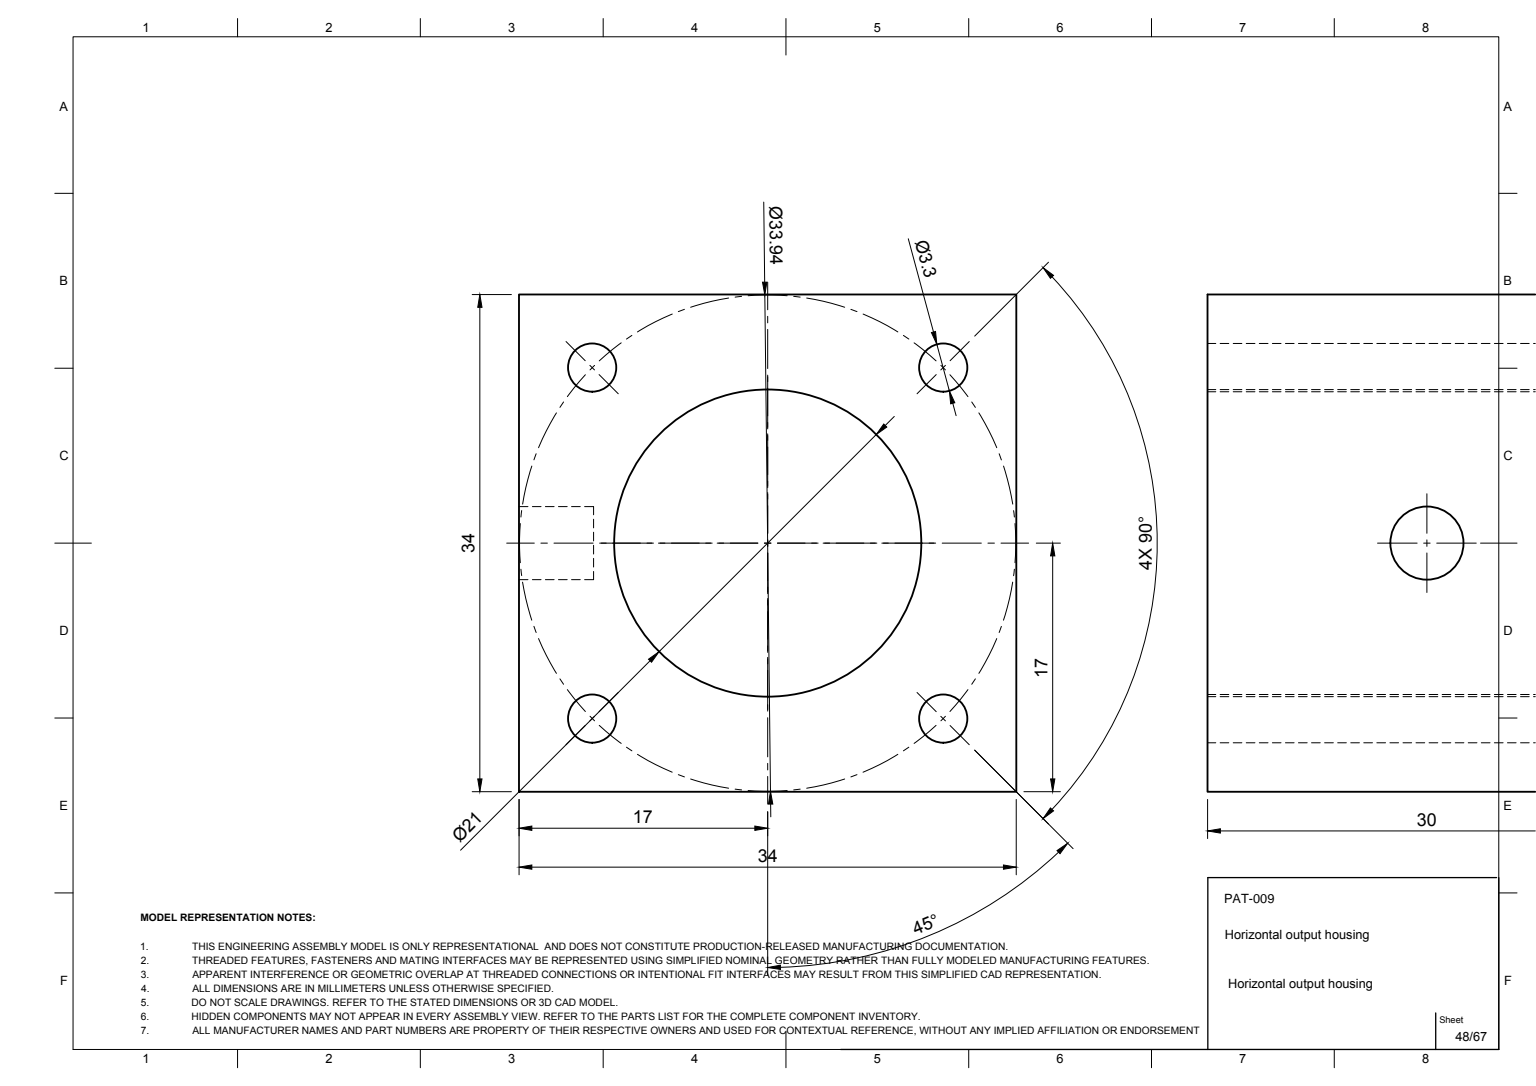
ISO-10303-21;
HEADER;
/* Generated by software containing ST-Developer
 * from STEP Tools, Inc. (www.steptools.com) 
 */

FILE_DESCRIPTION(
/* description */ ('Bell-crank linkage with push rods'),
/* implementation_level */ '2;1');

FILE_NAME(
/* name */ 'Horizontal output housing.step',
/* time_stamp */ '2026-10-28T03:25:15-07:00',
/* author */ (''),
/* organization */ (''),
/* preprocessor_version */ 'ST-DEVELOPER v20.2',
/* originating_system */ 'Autodesk Translation Framework v15.17.0.0',
/* authorisation */ '');

FILE_SCHEMA (('AUTOMOTIVE_DESIGN { 1 0 10303 214 3 1 1 }'));
ENDSEC;

DATA;
#10=MECHANICAL_DESIGN_GEOMETRIC_PRESENTATION_REPRESENTATION('',(#649),#16678);
#533=SHAPE_REPRESENTATION_RELATIONSHIP('SRR','None',#16954,#587);
#587=ADVANCED_BREP_SHAPE_REPRESENTATION('',(#709),#16659);
#649=STYLED_ITEM('',(#17270),#709);
#709=MANIFOLD_SOLID_BREP('Body1',#8841);
#874=FACE_BOUND('',#2296,.T.);
#875=FACE_BOUND('',#2297,.T.);
#876=FACE_BOUND('',#2298,.T.);
#877=FACE_BOUND('',#2299,.T.);
#878=FACE_BOUND('',#2300,.T.);
#879=FACE_BOUND('',#2303,.T.);
#880=FACE_BOUND('',#2304,.T.);
#881=FACE_BOUND('',#2305,.T.);
#882=FACE_BOUND('',#2306,.T.);
#883=FACE_BOUND('',#2307,.T.);
#884=FACE_BOUND('',#2309,.T.);
#1159=PLANE('',#10239);
#1160=PLANE('',#10255);
#1161=PLANE('',#10256);
#1162=PLANE('',#10257);
#1163=PLANE('',#10258);
#1164=PLANE('',#10259);
#1165=PLANE('',#10260);
#1616=FACE_OUTER_BOUND('',#2287,.T.);
#1617=FACE_OUTER_BOUND('',#2288,.T.);
#1618=FACE_OUTER_BOUND('',#2289,.T.);
#1619=FACE_OUTER_BOUND('',#2290,.T.);
#1620=FACE_OUTER_BOUND('',#2291,.T.);
#1621=FACE_OUTER_BOUND('',#2292,.T.);
#1622=FACE_OUTER_BOUND('',#2293,.T.);
#1623=FACE_OUTER_BOUND('',#2294,.T.);
#1624=FACE_OUTER_BOUND('',#2295,.T.);
#1625=FACE_OUTER_BOUND('',#2301,.T.);
#1626=FACE_OUTER_BOUND('',#2302,.T.);
#1627=FACE_OUTER_BOUND('',#2308,.T.);
#1628=FACE_OUTER_BOUND('',#2310,.T.);
#2287=EDGE_LOOP('',(#7455,#7456,#7457,#7458));
#2288=EDGE_LOOP('',(#7459));
#2289=EDGE_LOOP('',(#7460,#7461,#7462,#7463));
#2290=EDGE_LOOP('',(#7464,#7465,#7466,#7467));
#2291=EDGE_LOOP('',(#7468,#7469,#7470,#7471));
#2292=EDGE_LOOP('',(#7472,#7473,#7474,#7475));
#2293=EDGE_LOOP('',(#7476,#7477,#7478,#7479));
#2294=EDGE_LOOP('',(#7480,#7481,#7482,#7483));
#2295=EDGE_LOOP('',(#7484,#7485,#7486,#7487));
#2296=EDGE_LOOP('',(#7488));
#2297=EDGE_LOOP('',(#7489));
#2298=EDGE_LOOP('',(#7490));
#2299=EDGE_LOOP('',(#7491));
#2300=EDGE_LOOP('',(#7492));
#2301=EDGE_LOOP('',(#7493,#7494,#7495,#7496));
#2302=EDGE_LOOP('',(#7497,#7498,#7499,#7500));
#2303=EDGE_LOOP('',(#7501));
#2304=EDGE_LOOP('',(#7502));
#2305=EDGE_LOOP('',(#7503));
#2306=EDGE_LOOP('',(#7504));
#2307=EDGE_LOOP('',(#7505));
#2308=EDGE_LOOP('',(#7506,#7507,#7508,#7509));
#2309=EDGE_LOOP('',(#7510));
#2310=EDGE_LOOP('',(#7511,#7512,#7513,#7514));
#2908=LINE('',#15785,#3457);
#2909=LINE('',#15792,#3458);
#2910=LINE('',#15798,#3459);
#2911=LINE('',#15804,#3460);
#2912=LINE('',#15810,#3461);
#2913=LINE('',#15816,#3462);
#2914=LINE('',#15821,#3463);
#2915=LINE('',#15823,#3464);
#2916=LINE('',#15825,#3465);
#2917=LINE('',#15826,#3466);
#2918=LINE('',#15829,#3467);
#2919=LINE('',#15831,#3468);
#2920=LINE('',#15832,#3469);
#2921=LINE('',#15835,#3470);
#2922=LINE('',#15837,#3471);
#2923=LINE('',#15838,#3472);
#2924=LINE('',#15840,#3473);
#2925=LINE('',#15841,#3474);
#3457=VECTOR('',#12574,0.25);
#3458=VECTOR('',#12583,0.165);
#3459=VECTOR('',#12590,0.165);
#3460=VECTOR('',#12597,0.165);
#3461=VECTOR('',#12604,0.165);
#3462=VECTOR('',#12611,1.05);
#3463=VECTOR('',#12616,1.);
#3464=VECTOR('',#12617,1.);
#3465=VECTOR('',#12618,1.);
#3466=VECTOR('',#12619,1.);
#3467=VECTOR('',#12622,1.);
#3468=VECTOR('',#12623,1.);
#3469=VECTOR('',#12624,1.);
#3470=VECTOR('',#12627,1.);
#3471=VECTOR('',#12628,1.);
#3472=VECTOR('',#12629,1.);
#3473=VECTOR('',#12632,1.);
#3474=VECTOR('',#12633,1.);
#3987=CIRCLE('',#10237,0.25);
#3988=CIRCLE('',#10238,0.25);
#3989=CIRCLE('',#10241,0.165);
#3990=CIRCLE('',#10242,0.165);
#3991=CIRCLE('',#10244,0.165);
#3992=CIRCLE('',#10245,0.165);
#3993=CIRCLE('',#10247,0.165);
#3994=CIRCLE('',#10248,0.165);
#3995=CIRCLE('',#10250,0.165);
#3996=CIRCLE('',#10251,0.165);
#3997=CIRCLE('',#10253,1.05);
#3998=CIRCLE('',#10254,1.05);
#4630=VERTEX_POINT('',#15782);
#4631=VERTEX_POINT('',#15784);
#4632=VERTEX_POINT('',#15789);
#4633=VERTEX_POINT('',#15791);
#4634=VERTEX_POINT('',#15795);
#4635=VERTEX_POINT('',#15797);
#4636=VERTEX_POINT('',#15801);
#4637=VERTEX_POINT('',#15803);
#4638=VERTEX_POINT('',#15807);
#4639=VERTEX_POINT('',#15809);
#4640=VERTEX_POINT('',#15813);
#4641=VERTEX_POINT('',#15815);
#4642=VERTEX_POINT('',#15819);
#4643=VERTEX_POINT('',#15820);
#4644=VERTEX_POINT('',#15822);
#4645=VERTEX_POINT('',#15824);
#4646=VERTEX_POINT('',#15828);
#4647=VERTEX_POINT('',#15830);
#4648=VERTEX_POINT('',#15834);
#4649=VERTEX_POINT('',#15836);
#5605=EDGE_CURVE('',#4630,#4630,#3987,.T.);
#5606=EDGE_CURVE('',#4630,#4631,#2908,.T.);
#5607=EDGE_CURVE('',#4631,#4631,#3988,.T.);
#5608=EDGE_CURVE('',#4632,#4632,#3989,.T.);
#5609=EDGE_CURVE('',#4632,#4633,#2909,.T.);
#5610=EDGE_CURVE('',#4633,#4633,#3990,.T.);
#5611=EDGE_CURVE('',#4634,#4634,#3991,.T.);
#5612=EDGE_CURVE('',#4634,#4635,#2910,.T.);
#5613=EDGE_CURVE('',#4635,#4635,#3992,.T.);
#5614=EDGE_CURVE('',#4636,#4636,#3993,.T.);
#5615=EDGE_CURVE('',#4636,#4637,#2911,.T.);
#5616=EDGE_CURVE('',#4637,#4637,#3994,.T.);
#5617=EDGE_CURVE('',#4638,#4638,#3995,.T.);
#5618=EDGE_CURVE('',#4638,#4639,#2912,.T.);
#5619=EDGE_CURVE('',#4639,#4639,#3996,.T.);
#5620=EDGE_CURVE('',#4640,#4640,#3997,.T.);
#5621=EDGE_CURVE('',#4640,#4641,#2913,.T.);
#5622=EDGE_CURVE('',#4641,#4641,#3998,.T.);
#5623=EDGE_CURVE('',#4642,#4643,#2914,.T.);
#5624=EDGE_CURVE('',#4643,#4644,#2915,.T.);
#5625=EDGE_CURVE('',#4645,#4644,#2916,.T.);
#5626=EDGE_CURVE('',#4642,#4645,#2917,.T.);
#5627=EDGE_CURVE('',#4646,#4642,#2918,.T.);
#5628=EDGE_CURVE('',#4647,#4645,#2919,.T.);
#5629=EDGE_CURVE('',#4646,#4647,#2920,.T.);
#5630=EDGE_CURVE('',#4648,#4646,#2921,.T.);
#5631=EDGE_CURVE('',#4649,#4647,#2922,.T.);
#5632=EDGE_CURVE('',#4648,#4649,#2923,.T.);
#5633=EDGE_CURVE('',#4643,#4648,#2924,.T.);
#5634=EDGE_CURVE('',#4644,#4649,#2925,.T.);
#7455=ORIENTED_EDGE('',*,*,#5605,.F.);
#7456=ORIENTED_EDGE('',*,*,#5606,.T.);
#7457=ORIENTED_EDGE('',*,*,#5607,.F.);
#7458=ORIENTED_EDGE('',*,*,#5606,.F.);
#7459=ORIENTED_EDGE('',*,*,#5605,.T.);
#7460=ORIENTED_EDGE('',*,*,#5608,.F.);
#7461=ORIENTED_EDGE('',*,*,#5609,.T.);
#7462=ORIENTED_EDGE('',*,*,#5610,.F.);
#7463=ORIENTED_EDGE('',*,*,#5609,.F.);
#7464=ORIENTED_EDGE('',*,*,#5611,.F.);
#7465=ORIENTED_EDGE('',*,*,#5612,.T.);
#7466=ORIENTED_EDGE('',*,*,#5613,.F.);
#7467=ORIENTED_EDGE('',*,*,#5612,.F.);
#7468=ORIENTED_EDGE('',*,*,#5614,.F.);
#7469=ORIENTED_EDGE('',*,*,#5615,.T.);
#7470=ORIENTED_EDGE('',*,*,#5616,.F.);
#7471=ORIENTED_EDGE('',*,*,#5615,.F.);
#7472=ORIENTED_EDGE('',*,*,#5617,.F.);
#7473=ORIENTED_EDGE('',*,*,#5618,.T.);
#7474=ORIENTED_EDGE('',*,*,#5619,.F.);
#7475=ORIENTED_EDGE('',*,*,#5618,.F.);
#7476=ORIENTED_EDGE('',*,*,#5620,.F.);
#7477=ORIENTED_EDGE('',*,*,#5621,.T.);
#7478=ORIENTED_EDGE('',*,*,#5622,.F.);
#7479=ORIENTED_EDGE('',*,*,#5621,.F.);
#7480=ORIENTED_EDGE('',*,*,#5623,.T.);
#7481=ORIENTED_EDGE('',*,*,#5624,.T.);
#7482=ORIENTED_EDGE('',*,*,#5625,.F.);
#7483=ORIENTED_EDGE('',*,*,#5626,.F.);
#7484=ORIENTED_EDGE('',*,*,#5627,.T.);
#7485=ORIENTED_EDGE('',*,*,#5626,.T.);
#7486=ORIENTED_EDGE('',*,*,#5628,.F.);
#7487=ORIENTED_EDGE('',*,*,#5629,.F.);
#7488=ORIENTED_EDGE('',*,*,#5622,.T.);
#7489=ORIENTED_EDGE('',*,*,#5619,.T.);
#7490=ORIENTED_EDGE('',*,*,#5616,.T.);
#7491=ORIENTED_EDGE('',*,*,#5613,.T.);
#7492=ORIENTED_EDGE('',*,*,#5610,.T.);
#7493=ORIENTED_EDGE('',*,*,#5630,.T.);
#7494=ORIENTED_EDGE('',*,*,#5629,.T.);
#7495=ORIENTED_EDGE('',*,*,#5631,.F.);
#7496=ORIENTED_EDGE('',*,*,#5632,.F.);
#7497=ORIENTED_EDGE('',*,*,#5633,.T.);
#7498=ORIENTED_EDGE('',*,*,#5632,.T.);
#7499=ORIENTED_EDGE('',*,*,#5634,.F.);
#7500=ORIENTED_EDGE('',*,*,#5624,.F.);
#7501=ORIENTED_EDGE('',*,*,#5620,.T.);
#7502=ORIENTED_EDGE('',*,*,#5617,.T.);
#7503=ORIENTED_EDGE('',*,*,#5614,.T.);
#7504=ORIENTED_EDGE('',*,*,#5611,.T.);
#7505=ORIENTED_EDGE('',*,*,#5608,.T.);
#7506=ORIENTED_EDGE('',*,*,#5634,.T.);
#7507=ORIENTED_EDGE('',*,*,#5631,.T.);
#7508=ORIENTED_EDGE('',*,*,#5628,.T.);
#7509=ORIENTED_EDGE('',*,*,#5625,.T.);
#7510=ORIENTED_EDGE('',*,*,#5607,.T.);
#7511=ORIENTED_EDGE('',*,*,#5633,.F.);
#7512=ORIENTED_EDGE('',*,*,#5623,.F.);
#7513=ORIENTED_EDGE('',*,*,#5627,.F.);
#7514=ORIENTED_EDGE('',*,*,#5630,.F.);
#8210=CYLINDRICAL_SURFACE('',#10236,0.25);
#8211=CYLINDRICAL_SURFACE('',#10240,0.165);
#8212=CYLINDRICAL_SURFACE('',#10243,0.165);
#8213=CYLINDRICAL_SURFACE('',#10246,0.165);
#8214=CYLINDRICAL_SURFACE('',#10249,0.165);
#8215=CYLINDRICAL_SURFACE('',#10252,1.05);
#8641=ADVANCED_FACE('',(#1616),#8210,.F.);
#8642=ADVANCED_FACE('',(#1617),#1159,.T.);
#8643=ADVANCED_FACE('',(#1618),#8211,.F.);
#8644=ADVANCED_FACE('',(#1619),#8212,.F.);
#8645=ADVANCED_FACE('',(#1620),#8213,.F.);
#8646=ADVANCED_FACE('',(#1621),#8214,.F.);
#8647=ADVANCED_FACE('',(#1622),#8215,.F.);
#8648=ADVANCED_FACE('',(#1623),#1160,.T.);
#8649=ADVANCED_FACE('',(#1624,#874,#875,#876,#877,#878),#1161,.T.);
#8650=ADVANCED_FACE('',(#1625),#1162,.T.);
#8651=ADVANCED_FACE('',(#1626,#879,#880,#881,#882,#883),#1163,.T.);
#8652=ADVANCED_FACE('',(#1627,#884),#1164,.T.);
#8653=ADVANCED_FACE('',(#1628),#1165,.F.);
#8841=CLOSED_SHELL('',(#8641,#8642,#8643,#8644,#8645,#8646,#8647,#8648,
#8649,#8650,#8651,#8652,#8653));
#10235=AXIS2_PLACEMENT_3D('',#15780,#12568,#12569);
#10236=AXIS2_PLACEMENT_3D('',#15781,#12570,#12571);
#10237=AXIS2_PLACEMENT_3D('',#15783,#12572,#12573);
#10238=AXIS2_PLACEMENT_3D('',#15786,#12575,#12576);
#10239=AXIS2_PLACEMENT_3D('',#15787,#12577,#12578);
#10240=AXIS2_PLACEMENT_3D('',#15788,#12579,#12580);
#10241=AXIS2_PLACEMENT_3D('',#15790,#12581,#12582);
#10242=AXIS2_PLACEMENT_3D('',#15793,#12584,#12585);
#10243=AXIS2_PLACEMENT_3D('',#15794,#12586,#12587);
#10244=AXIS2_PLACEMENT_3D('',#15796,#12588,#12589);
#10245=AXIS2_PLACEMENT_3D('',#15799,#12591,#12592);
#10246=AXIS2_PLACEMENT_3D('',#15800,#12593,#12594);
#10247=AXIS2_PLACEMENT_3D('',#15802,#12595,#12596);
#10248=AXIS2_PLACEMENT_3D('',#15805,#12598,#12599);
#10249=AXIS2_PLACEMENT_3D('',#15806,#12600,#12601);
#10250=AXIS2_PLACEMENT_3D('',#15808,#12602,#12603);
#10251=AXIS2_PLACEMENT_3D('',#15811,#12605,#12606);
#10252=AXIS2_PLACEMENT_3D('',#15812,#12607,#12608);
#10253=AXIS2_PLACEMENT_3D('',#15814,#12609,#12610);
#10254=AXIS2_PLACEMENT_3D('',#15817,#12612,#12613);
#10255=AXIS2_PLACEMENT_3D('',#15818,#12614,#12615);
#10256=AXIS2_PLACEMENT_3D('',#15827,#12620,#12621);
#10257=AXIS2_PLACEMENT_3D('',#15833,#12625,#12626);
#10258=AXIS2_PLACEMENT_3D('',#15839,#12630,#12631);
#10259=AXIS2_PLACEMENT_3D('',#15842,#12634,#12635);
#10260=AXIS2_PLACEMENT_3D('',#15843,#12636,#12637);
#12568=DIRECTION('axis',(0.,0.,1.));
#12569=DIRECTION('refdir',(1.,0.,0.));
#12570=DIRECTION('center_axis',(0.,0.,1.));
#12571=DIRECTION('ref_axis',(1.,0.,0.));
#12572=DIRECTION('center_axis',(0.,0.,1.));
#12573=DIRECTION('ref_axis',(1.,0.,0.));
#12574=DIRECTION('',(0.,0.,1.));
#12575=DIRECTION('center_axis',(0.,0.,-1.));
#12576=DIRECTION('ref_axis',(1.,0.,0.));
#12577=DIRECTION('center_axis',(0.,0.,1.));
#12578=DIRECTION('ref_axis',(1.,0.,0.));
#12579=DIRECTION('center_axis',(1.,0.,0.));
#12580=DIRECTION('ref_axis',(0.,0.,-1.));
#12581=DIRECTION('center_axis',(1.,0.,0.));
#12582=DIRECTION('ref_axis',(0.,0.,-1.));
#12583=DIRECTION('',(1.,0.,0.));
#12584=DIRECTION('center_axis',(-1.,0.,0.));
#12585=DIRECTION('ref_axis',(0.,0.,-1.));
#12586=DIRECTION('center_axis',(1.,0.,0.));
#12587=DIRECTION('ref_axis',(0.,0.,-1.));
#12588=DIRECTION('center_axis',(1.,0.,0.));
#12589=DIRECTION('ref_axis',(0.,0.,-1.));
#12590=DIRECTION('',(1.,0.,0.));
#12591=DIRECTION('center_axis',(-1.,0.,0.));
#12592=DIRECTION('ref_axis',(0.,0.,-1.));
#12593=DIRECTION('center_axis',(1.,0.,0.));
#12594=DIRECTION('ref_axis',(0.,0.,-1.));
#12595=DIRECTION('center_axis',(1.,0.,0.));
#12596=DIRECTION('ref_axis',(0.,0.,-1.));
#12597=DIRECTION('',(1.,0.,0.));
#12598=DIRECTION('center_axis',(-1.,0.,0.));
#12599=DIRECTION('ref_axis',(0.,0.,-1.));
#12600=DIRECTION('center_axis',(1.,0.,0.));
#12601=DIRECTION('ref_axis',(0.,0.,-1.));
#12602=DIRECTION('center_axis',(1.,0.,0.));
#12603=DIRECTION('ref_axis',(0.,0.,-1.));
#12604=DIRECTION('',(1.,0.,0.));
#12605=DIRECTION('center_axis',(-1.,0.,0.));
#12606=DIRECTION('ref_axis',(0.,0.,-1.));
#12607=DIRECTION('center_axis',(1.,0.,0.));
#12608=DIRECTION('ref_axis',(0.,0.,-1.));
#12609=DIRECTION('center_axis',(1.,0.,0.));
#12610=DIRECTION('ref_axis',(0.,0.,-1.));
#12611=DIRECTION('',(1.,0.,0.));
#12612=DIRECTION('center_axis',(-1.,0.,0.));
#12613=DIRECTION('ref_axis',(0.,0.,-1.));
#12614=DIRECTION('center_axis',(0.,1.,0.));
#12615=DIRECTION('ref_axis',(-1.,0.,0.));
#12616=DIRECTION('',(-1.,0.,0.));
#12617=DIRECTION('',(0.,0.,1.));
#12618=DIRECTION('',(-1.,0.,0.));
#12619=DIRECTION('',(0.,0.,1.));
#12620=DIRECTION('center_axis',(1.,0.,0.));
#12621=DIRECTION('ref_axis',(0.,1.,0.));
#12622=DIRECTION('',(0.,1.,0.));
#12623=DIRECTION('',(0.,1.,0.));
#12624=DIRECTION('',(0.,0.,1.));
#12625=DIRECTION('center_axis',(0.,-1.,0.));
#12626=DIRECTION('ref_axis',(1.,0.,0.));
#12627=DIRECTION('',(1.,0.,0.));
#12628=DIRECTION('',(1.,0.,0.));
#12629=DIRECTION('',(0.,0.,1.));
#12630=DIRECTION('center_axis',(-1.,0.,0.));
#12631=DIRECTION('ref_axis',(0.,-1.,0.));
#12632=DIRECTION('',(0.,-1.,0.));
#12633=DIRECTION('',(0.,-1.,0.));
#12634=DIRECTION('center_axis',(0.,0.,1.));
#12635=DIRECTION('ref_axis',(1.,0.,0.));
#12636=DIRECTION('center_axis',(0.,0.,1.));
#12637=DIRECTION('ref_axis',(1.,0.,0.));
#15780=CARTESIAN_POINT('',(0.,0.,0.));
#15781=CARTESIAN_POINT('Origin',(10.,2.,5.19));
#15782=CARTESIAN_POINT('',(9.75,2.,5.19));
#15783=CARTESIAN_POINT('Origin',(10.,2.,5.19));
#15784=CARTESIAN_POINT('',(9.75,2.,5.7));
#15785=CARTESIAN_POINT('',(9.75,2.,5.19));
#15786=CARTESIAN_POINT('Origin',(10.,2.,5.7));
#15787=CARTESIAN_POINT('Origin',(10.,2.,5.19));
#15788=CARTESIAN_POINT('Origin',(8.4,3.2,2.8));
#15789=CARTESIAN_POINT('',(8.5,3.2,2.965));
#15790=CARTESIAN_POINT('Origin',(8.5,3.2,2.8));
#15791=CARTESIAN_POINT('',(11.5,3.2,2.965));
#15792=CARTESIAN_POINT('',(8.4,3.2,2.965));
#15793=CARTESIAN_POINT('Origin',(11.5,3.2,2.8));
#15794=CARTESIAN_POINT('Origin',(8.4,0.8,5.2));
#15795=CARTESIAN_POINT('',(8.5,0.8,5.365));
#15796=CARTESIAN_POINT('Origin',(8.5,0.8,5.2));
#15797=CARTESIAN_POINT('',(11.5,0.8,5.365));
#15798=CARTESIAN_POINT('',(8.4,0.8,5.365));
#15799=CARTESIAN_POINT('Origin',(11.5,0.8,5.2));
#15800=CARTESIAN_POINT('Origin',(8.4,0.8,2.8));
#15801=CARTESIAN_POINT('',(8.5,0.8,2.965));
#15802=CARTESIAN_POINT('Origin',(8.5,0.8,2.8));
#15803=CARTESIAN_POINT('',(11.5,0.8,2.965));
#15804=CARTESIAN_POINT('',(8.4,0.8,2.965));
#15805=CARTESIAN_POINT('Origin',(11.5,0.8,2.8));
#15806=CARTESIAN_POINT('Origin',(8.4,3.2,5.2));
#15807=CARTESIAN_POINT('',(8.5,3.2,5.365));
#15808=CARTESIAN_POINT('Origin',(8.5,3.2,5.2));
#15809=CARTESIAN_POINT('',(11.5,3.2,5.365));
#15810=CARTESIAN_POINT('',(8.4,3.2,5.365));
#15811=CARTESIAN_POINT('Origin',(11.5,3.2,5.2));
#15812=CARTESIAN_POINT('Origin',(8.4,2.,4.));
#15813=CARTESIAN_POINT('',(8.5,2.,5.05));
#15814=CARTESIAN_POINT('Origin',(8.5,2.,4.));
#15815=CARTESIAN_POINT('',(11.5,2.,5.05));
#15816=CARTESIAN_POINT('',(8.4,2.,5.05));
#15817=CARTESIAN_POINT('Origin',(11.5,2.,4.));
#15818=CARTESIAN_POINT('Origin',(11.5,3.7,2.3));
#15819=CARTESIAN_POINT('',(11.5,3.7,2.3));
#15820=CARTESIAN_POINT('',(8.5,3.7,2.3));
#15821=CARTESIAN_POINT('',(11.5,3.7,2.3));
#15822=CARTESIAN_POINT('',(8.5,3.7,5.7));
#15823=CARTESIAN_POINT('',(8.5,3.7,2.3));
#15824=CARTESIAN_POINT('',(11.5,3.7,5.7));
#15825=CARTESIAN_POINT('',(11.5,3.7,5.7));
#15826=CARTESIAN_POINT('',(11.5,3.7,2.3));
#15827=CARTESIAN_POINT('Origin',(11.5,0.3,2.3));
#15828=CARTESIAN_POINT('',(11.5,0.3,2.3));
#15829=CARTESIAN_POINT('',(11.5,0.3,2.3));
#15830=CARTESIAN_POINT('',(11.5,0.3,5.7));
#15831=CARTESIAN_POINT('',(11.5,0.3,5.7));
#15832=CARTESIAN_POINT('',(11.5,0.3,2.3));
#15833=CARTESIAN_POINT('Origin',(8.5,0.3,2.3));
#15834=CARTESIAN_POINT('',(8.5,0.3,2.3));
#15835=CARTESIAN_POINT('',(8.5,0.3,2.3));
#15836=CARTESIAN_POINT('',(8.5,0.3,5.7));
#15837=CARTESIAN_POINT('',(8.5,0.3,5.7));
#15838=CARTESIAN_POINT('',(8.5,0.3,2.3));
#15839=CARTESIAN_POINT('Origin',(8.5,3.7,2.3));
#15840=CARTESIAN_POINT('',(8.5,3.7,2.3));
#15841=CARTESIAN_POINT('',(8.5,3.7,5.7));
#15842=CARTESIAN_POINT('Origin',(10.,2.,5.7));
#15843=CARTESIAN_POINT('Origin',(10.,2.,2.3));
#16595=UNCERTAINTY_MEASURE_WITH_UNIT(LENGTH_MEASURE(0.001),#16679,
'DISTANCE_ACCURACY_VALUE',
'Maximum model space distance between geometric entities at asserted c
onnectivities');
#16614=UNCERTAINTY_MEASURE_WITH_UNIT(LENGTH_MEASURE(0.001),#16679,
'DISTANCE_ACCURACY_VALUE',
'Maximum model space distance between geometric entities at asserted c
onnectivities');
#16659=(
GEOMETRIC_REPRESENTATION_CONTEXT(3)
GLOBAL_UNCERTAINTY_ASSIGNED_CONTEXT((#16595))
GLOBAL_UNIT_ASSIGNED_CONTEXT((#16679,#16681,#16682))
REPRESENTATION_CONTEXT('','3D')
);
#16678=(
GEOMETRIC_REPRESENTATION_CONTEXT(3)
GLOBAL_UNCERTAINTY_ASSIGNED_CONTEXT((#16614))
GLOBAL_UNIT_ASSIGNED_CONTEXT((#16679,#16681,#16682))
REPRESENTATION_CONTEXT('','3D')
);
#16679=(
LENGTH_UNIT()
NAMED_UNIT(*)
SI_UNIT(.CENTI.,.METRE.)
);
#16681=(
NAMED_UNIT(*)
PLANE_ANGLE_UNIT()
SI_UNIT($,.RADIAN.)
);
#16682=(
NAMED_UNIT(*)
SI_UNIT($,.STERADIAN.)
SOLID_ANGLE_UNIT()
);
#16727=SHAPE_DEFINITION_REPRESENTATION(#16801,#16954);
#16801=PRODUCT_DEFINITION_SHAPE('',$,#17018);
#16954=SHAPE_REPRESENTATION('',(#10235),#16659);
#16973=PRODUCT_DEFINITION_CONTEXT('part definition',#17164,'design');
#17018=PRODUCT_DEFINITION('Horizontal output housing',
'Horizontal output housing',#17081,#16973);
#17081=PRODUCT_DEFINITION_FORMATION('',$,#17210);
#17164=APPLICATION_CONTEXT(
'Core Data for Automotive Mechanical Design Process');
#17165=PRODUCT_CONTEXT('part definition',#17164,'mechanical');
#17210=PRODUCT('Horizontal output housing','Horizontal output housing',
'Horizontal output housing',(#17165));
#17264=COLOUR_RGB('Dark Blue',0.08,0.2,0.34);
#17265=FILL_AREA_STYLE_COLOUR('',#17264);
#17266=FILL_AREA_STYLE('',(#17265));
#17267=SURFACE_STYLE_FILL_AREA(#17266);
#17268=SURFACE_SIDE_STYLE('',(#17267));
#17269=SURFACE_STYLE_USAGE(.BOTH.,#17268);
#17270=PRESENTATION_STYLE_ASSIGNMENT((#17269));
ENDSEC;
END-ISO-10303-21;
